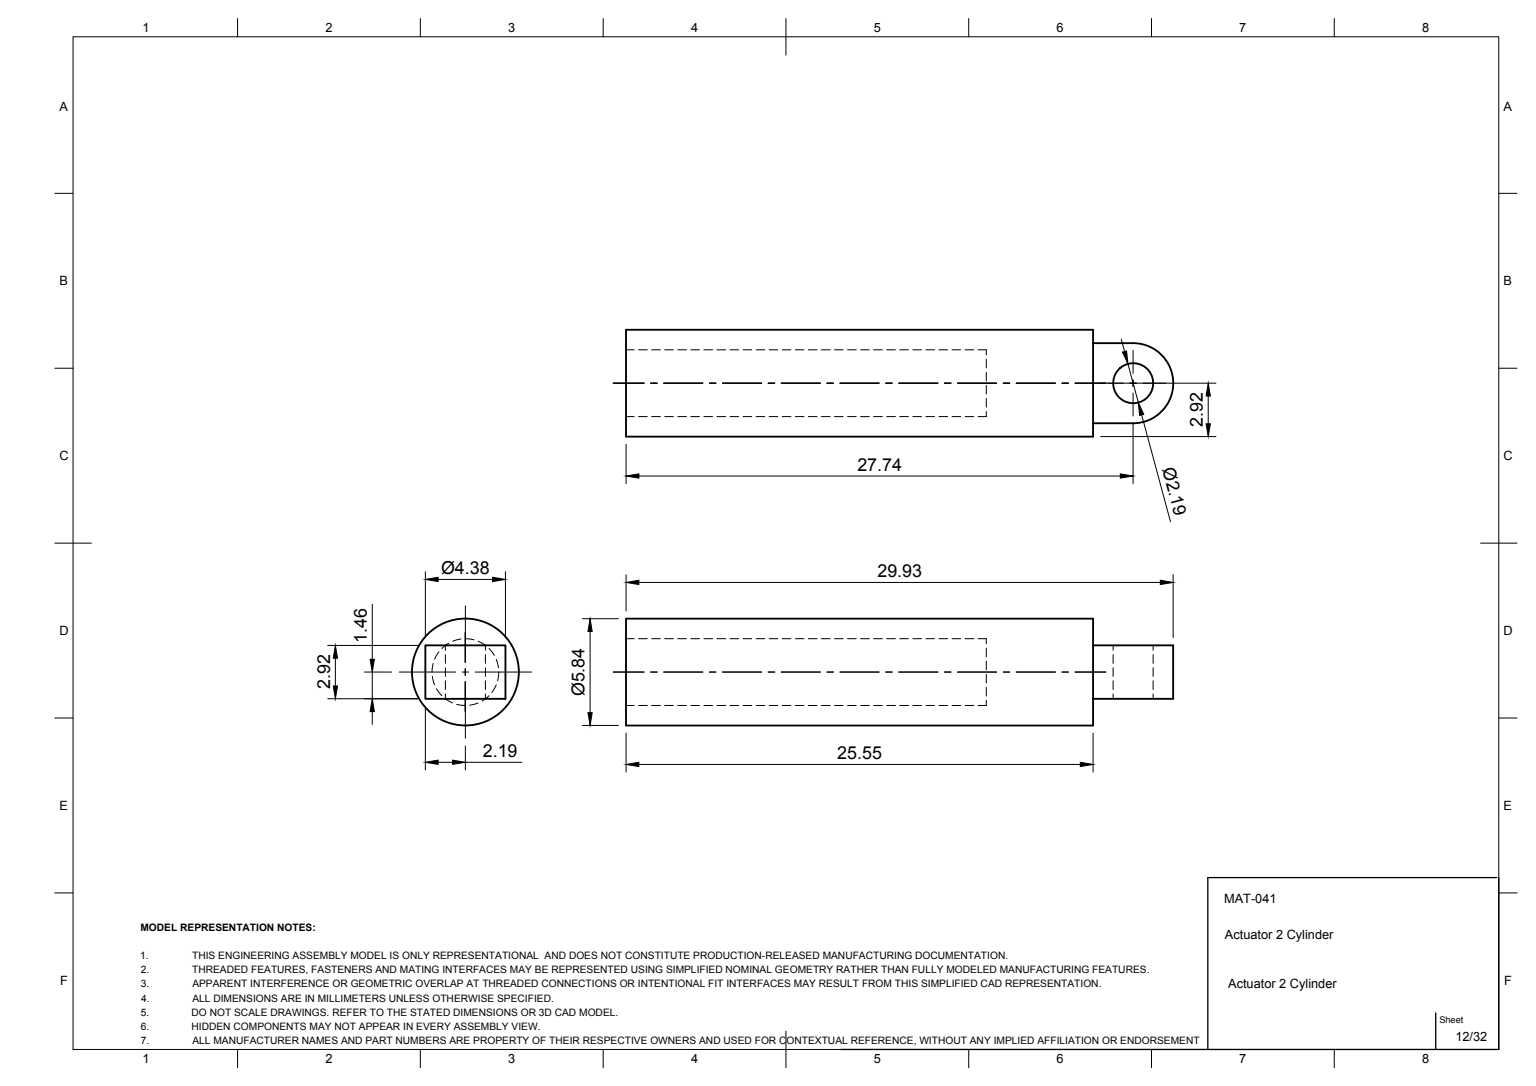
ISO-10303-21;
HEADER;
/* Generated by software containing ST-Developer
 * from STEP Tools, Inc. (www.steptools.com) 
 */

FILE_DESCRIPTION(
/* description */ ('STEP AP214'),
/* implementation_level */ '2;1');

FILE_NAME(
/* name */ 'Actuator 2 Cylinder.step',
/* time_stamp */ '2026-11-14T21:57:47-08:00',
/* author */ (''),
/* organization */ (''),
/* preprocessor_version */ 'ST-DEVELOPER v20.2',
/* originating_system */ 'Autodesk Translation Framework v15.17.0.0',
/* authorisation */ '');

FILE_SCHEMA (('AUTOMOTIVE_DESIGN { 1 0 10303 214 3 1 1 }'));
ENDSEC;

DATA;
#10=MECHANICAL_DESIGN_GEOMETRIC_PRESENTATION_REPRESENTATION('',(#252),#13199);
#216=SHAPE_REPRESENTATION_RELATIONSHIP('SRR','None',#13285,#234);
#234=ADVANCED_BREP_SHAPE_REPRESENTATION('',(#270),#13181);
#252=STYLED_ITEM('',(#13409),#270);
#270=MANIFOLD_SOLID_BREP('Body1',#6847);
#324=FACE_BOUND('',#2433,.T.);
#325=FACE_BOUND('',#2435,.T.);
#326=FACE_BOUND('',#2437,.T.);
#327=FACE_BOUND('',#2440,.T.);
#485=PLANE('',#7464);
#486=PLANE('',#7465);
#487=PLANE('',#7466);
#488=PLANE('',#7468);
#489=PLANE('',#7469);
#490=PLANE('',#7471);
#491=PLANE('',#7473);
#860=LINE('',#11592,#1378);
#861=LINE('',#11598,#1379);
#862=LINE('',#11604,#1380);
#863=LINE('',#11609,#1381);
#864=LINE('',#11611,#1382);
#865=LINE('',#11613,#1383);
#866=LINE('',#11614,#1384);
#867=LINE('',#11620,#1385);
#868=LINE('',#11621,#1386);
#869=LINE('',#11624,#1387);
#870=LINE('',#11625,#1388);
#871=LINE('',#11628,#1389);
#872=LINE('',#11631,#1390);
#1378=VECTOR('',#8873,1.825);
#1379=VECTOR('',#8880,1.095);
#1380=VECTOR('',#8887,2.92);
#1381=VECTOR('',#8892,1000.);
#1382=VECTOR('',#8893,1000.);
#1383=VECTOR('',#8894,1000.);
#1384=VECTOR('',#8895,1000.);
#1385=VECTOR('',#8902,1000.);
#1386=VECTOR('',#8903,1000.);
#1387=VECTOR('',#8906,1000.);
#1388=VECTOR('',#8907,1000.);
#1389=VECTOR('',#8910,1000.);
#1390=VECTOR('',#8915,1000.);
#1730=CYLINDRICAL_SURFACE('',#7455,1.825);
#1731=CYLINDRICAL_SURFACE('',#7458,1.095);
#1732=CYLINDRICAL_SURFACE('',#7461,2.92);
#1733=CYLINDRICAL_SURFACE('',#7472,2.19);
#1998=FACE_OUTER_BOUND('',#2429,.T.);
#1999=FACE_OUTER_BOUND('',#2430,.T.);
#2000=FACE_OUTER_BOUND('',#2431,.T.);
#2001=FACE_OUTER_BOUND('',#2432,.T.);
#2002=FACE_OUTER_BOUND('',#2434,.T.);
#2003=FACE_OUTER_BOUND('',#2436,.T.);
#2004=FACE_OUTER_BOUND('',#2438,.T.);
#2005=FACE_OUTER_BOUND('',#2439,.T.);
#2006=FACE_OUTER_BOUND('',#2441,.T.);
#2007=FACE_OUTER_BOUND('',#2442,.T.);
#2008=FACE_OUTER_BOUND('',#2443,.T.);
#2429=EDGE_LOOP('',(#5550,#5551,#5552,#5553));
#2430=EDGE_LOOP('',(#5554,#5555,#5556,#5557));
#2431=EDGE_LOOP('',(#5558,#5559,#5560,#5561));
#2432=EDGE_LOOP('',(#5562));
#2433=EDGE_LOOP('',(#5563,#5564,#5565,#5566));
#2434=EDGE_LOOP('',(#5567));
#2435=EDGE_LOOP('',(#5568));
#2436=EDGE_LOOP('',(#5569,#5570,#5571,#5572));
#2437=EDGE_LOOP('',(#5573));
#2438=EDGE_LOOP('',(#5574,#5575,#5576,#5577));
#2439=EDGE_LOOP('',(#5578,#5579,#5580,#5581));
#2440=EDGE_LOOP('',(#5582));
#2441=EDGE_LOOP('',(#5583,#5584,#5585,#5586));
#2442=EDGE_LOOP('',(#5587,#5588,#5589,#5590));
#2443=EDGE_LOOP('',(#5591));
#2861=CIRCLE('',#7456,1.825);
#2862=CIRCLE('',#7457,1.825);
#2863=CIRCLE('',#7459,1.095);
#2864=CIRCLE('',#7460,1.095);
#2865=CIRCLE('',#7462,2.92);
#2866=CIRCLE('',#7463,2.92);
#2867=CIRCLE('',#7467,2.19);
#2868=CIRCLE('',#7470,2.19);
#3318=VERTEX_POINT('',#11589);
#3319=VERTEX_POINT('',#11591);
#3320=VERTEX_POINT('',#11595);
#3321=VERTEX_POINT('',#11597);
#3322=VERTEX_POINT('',#11601);
#3323=VERTEX_POINT('',#11603);
#3324=VERTEX_POINT('',#11607);
#3325=VERTEX_POINT('',#11608);
#3326=VERTEX_POINT('',#11610);
#3327=VERTEX_POINT('',#11612);
#3328=VERTEX_POINT('',#11617);
#3329=VERTEX_POINT('',#11618);
#3330=VERTEX_POINT('',#11623);
#3331=VERTEX_POINT('',#11627);
#4112=EDGE_CURVE('',#3318,#3318,#2861,.T.);
#4113=EDGE_CURVE('',#3318,#3319,#860,.T.);
#4114=EDGE_CURVE('',#3319,#3319,#2862,.T.);
#4115=EDGE_CURVE('',#3320,#3320,#2863,.T.);
#4116=EDGE_CURVE('',#3320,#3321,#861,.T.);
#4117=EDGE_CURVE('',#3321,#3321,#2864,.T.);
#4118=EDGE_CURVE('',#3322,#3322,#2865,.T.);
#4119=EDGE_CURVE('',#3322,#3323,#862,.T.);
#4120=EDGE_CURVE('',#3323,#3323,#2866,.T.);
#4121=EDGE_CURVE('',#3324,#3325,#863,.T.);
#4122=EDGE_CURVE('',#3326,#3324,#864,.T.);
#4123=EDGE_CURVE('',#3327,#3326,#865,.T.);
#4124=EDGE_CURVE('',#3325,#3327,#866,.T.);
#4125=EDGE_CURVE('',#3328,#3329,#2867,.T.);
#4126=EDGE_CURVE('',#3329,#3324,#867,.T.);
#4127=EDGE_CURVE('',#3328,#3325,#868,.T.);
#4128=EDGE_CURVE('',#3330,#3327,#869,.T.);
#4129=EDGE_CURVE('',#3330,#3328,#870,.T.);
#4130=EDGE_CURVE('',#3331,#3326,#871,.T.);
#4131=EDGE_CURVE('',#3331,#3330,#2868,.T.);
#4132=EDGE_CURVE('',#3329,#3331,#872,.T.);
#5550=ORIENTED_EDGE('',*,*,#4112,.F.);
#5551=ORIENTED_EDGE('',*,*,#4113,.T.);
#5552=ORIENTED_EDGE('',*,*,#4114,.T.);
#5553=ORIENTED_EDGE('',*,*,#4113,.F.);
#5554=ORIENTED_EDGE('',*,*,#4115,.F.);
#5555=ORIENTED_EDGE('',*,*,#4116,.T.);
#5556=ORIENTED_EDGE('',*,*,#4117,.T.);
#5557=ORIENTED_EDGE('',*,*,#4116,.F.);
#5558=ORIENTED_EDGE('',*,*,#4118,.T.);
#5559=ORIENTED_EDGE('',*,*,#4119,.T.);
#5560=ORIENTED_EDGE('',*,*,#4120,.F.);
#5561=ORIENTED_EDGE('',*,*,#4119,.F.);
#5562=ORIENTED_EDGE('',*,*,#4118,.F.);
#5563=ORIENTED_EDGE('',*,*,#4121,.F.);
#5564=ORIENTED_EDGE('',*,*,#4122,.F.);
#5565=ORIENTED_EDGE('',*,*,#4123,.F.);
#5566=ORIENTED_EDGE('',*,*,#4124,.F.);
#5567=ORIENTED_EDGE('',*,*,#4120,.T.);
#5568=ORIENTED_EDGE('',*,*,#4114,.F.);
#5569=ORIENTED_EDGE('',*,*,#4125,.T.);
#5570=ORIENTED_EDGE('',*,*,#4126,.T.);
#5571=ORIENTED_EDGE('',*,*,#4121,.T.);
#5572=ORIENTED_EDGE('',*,*,#4127,.F.);
#5573=ORIENTED_EDGE('',*,*,#4115,.T.);
#5574=ORIENTED_EDGE('',*,*,#4128,.F.);
#5575=ORIENTED_EDGE('',*,*,#4129,.T.);
#5576=ORIENTED_EDGE('',*,*,#4127,.T.);
#5577=ORIENTED_EDGE('',*,*,#4124,.T.);
#5578=ORIENTED_EDGE('',*,*,#4130,.F.);
#5579=ORIENTED_EDGE('',*,*,#4131,.T.);
#5580=ORIENTED_EDGE('',*,*,#4128,.T.);
#5581=ORIENTED_EDGE('',*,*,#4123,.T.);
#5582=ORIENTED_EDGE('',*,*,#4117,.F.);
#5583=ORIENTED_EDGE('',*,*,#4126,.F.);
#5584=ORIENTED_EDGE('',*,*,#4132,.T.);
#5585=ORIENTED_EDGE('',*,*,#4130,.T.);
#5586=ORIENTED_EDGE('',*,*,#4122,.T.);
#5587=ORIENTED_EDGE('',*,*,#4129,.F.);
#5588=ORIENTED_EDGE('',*,*,#4131,.F.);
#5589=ORIENTED_EDGE('',*,*,#4132,.F.);
#5590=ORIENTED_EDGE('',*,*,#4125,.F.);
#5591=ORIENTED_EDGE('',*,*,#4112,.T.);
#6650=ADVANCED_FACE('',(#1998),#1730,.F.);
#6651=ADVANCED_FACE('',(#1999),#1731,.F.);
#6652=ADVANCED_FACE('',(#2000),#1732,.T.);
#6653=ADVANCED_FACE('',(#2001,#324),#485,.F.);
#6654=ADVANCED_FACE('',(#2002,#325),#486,.T.);
#6655=ADVANCED_FACE('',(#2003,#326),#487,.F.);
#6656=ADVANCED_FACE('',(#2004),#488,.F.);
#6657=ADVANCED_FACE('',(#2005,#327),#489,.F.);
#6658=ADVANCED_FACE('',(#2006),#490,.F.);
#6659=ADVANCED_FACE('',(#2007),#1733,.T.);
#6660=ADVANCED_FACE('',(#2008),#491,.T.);
#6847=CLOSED_SHELL('',(#6650,#6651,#6652,#6653,#6654,#6655,#6656,#6657,
#6658,#6659,#6660));
#7454=AXIS2_PLACEMENT_3D('',#11587,#8867,#8868);
#7455=AXIS2_PLACEMENT_3D('',#11588,#8869,#8870);
#7456=AXIS2_PLACEMENT_3D('',#11590,#8871,#8872);
#7457=AXIS2_PLACEMENT_3D('',#11593,#8874,#8875);
#7458=AXIS2_PLACEMENT_3D('',#11594,#8876,#8877);
#7459=AXIS2_PLACEMENT_3D('',#11596,#8878,#8879);
#7460=AXIS2_PLACEMENT_3D('',#11599,#8881,#8882);
#7461=AXIS2_PLACEMENT_3D('',#11600,#8883,#8884);
#7462=AXIS2_PLACEMENT_3D('',#11602,#8885,#8886);
#7463=AXIS2_PLACEMENT_3D('',#11605,#8888,#8889);
#7464=AXIS2_PLACEMENT_3D('',#11606,#8890,#8891);
#7465=AXIS2_PLACEMENT_3D('',#11615,#8896,#8897);
#7466=AXIS2_PLACEMENT_3D('',#11616,#8898,#8899);
#7467=AXIS2_PLACEMENT_3D('',#11619,#8900,#8901);
#7468=AXIS2_PLACEMENT_3D('',#11622,#8904,#8905);
#7469=AXIS2_PLACEMENT_3D('',#11626,#8908,#8909);
#7470=AXIS2_PLACEMENT_3D('',#11629,#8911,#8912);
#7471=AXIS2_PLACEMENT_3D('',#11630,#8913,#8914);
#7472=AXIS2_PLACEMENT_3D('',#11632,#8916,#8917);
#7473=AXIS2_PLACEMENT_3D('',#11633,#8918,#8919);
#8867=DIRECTION('axis',(0.,0.,1.));
#8868=DIRECTION('refdir',(1.,0.,0.));
#8869=DIRECTION('center_axis',(0.,0.,1.));
#8870=DIRECTION('ref_axis',(1.,0.,0.));
#8871=DIRECTION('center_axis',(0.,0.,1.));
#8872=DIRECTION('ref_axis',(1.,0.,0.));
#8873=DIRECTION('',(0.,0.,1.));
#8874=DIRECTION('center_axis',(0.,0.,1.));
#8875=DIRECTION('ref_axis',(1.,0.,0.));
#8876=DIRECTION('center_axis',(1.,-1.0842021724855E-16,0.));
#8877=DIRECTION('ref_axis',(1.0842021724855E-16,1.,0.));
#8878=DIRECTION('center_axis',(1.,-7.2280144832367E-17,0.));
#8879=DIRECTION('ref_axis',(7.2280144832367E-17,1.,0.));
#8880=DIRECTION('',(1.,-1.0842021724855E-16,0.));
#8881=DIRECTION('center_axis',(1.,-1.0842021724855E-16,0.));
#8882=DIRECTION('ref_axis',(1.0842021724855E-16,1.,0.));
#8883=DIRECTION('center_axis',(0.,0.,-1.));
#8884=DIRECTION('ref_axis',(-1.,0.,0.));
#8885=DIRECTION('center_axis',(0.,0.,1.));
#8886=DIRECTION('ref_axis',(1.,0.,0.));
#8887=DIRECTION('',(0.,0.,1.));
#8888=DIRECTION('center_axis',(0.,0.,1.));
#8889=DIRECTION('ref_axis',(1.,0.,0.));
#8890=DIRECTION('center_axis',(0.,0.,1.));
#8891=DIRECTION('ref_axis',(1.,0.,0.));
#8892=DIRECTION('',(7.2280144832367E-17,1.,0.));
#8893=DIRECTION('',(-1.,0.,0.));
#8894=DIRECTION('',(-1.44560289664734E-16,-1.,0.));
#8895=DIRECTION('',(1.,0.,0.));
#8896=DIRECTION('center_axis',(0.,0.,1.));
#8897=DIRECTION('ref_axis',(1.,0.,0.));
#8898=DIRECTION('center_axis',(1.,-7.2280144832367E-17,0.));
#8899=DIRECTION('ref_axis',(7.2280144832367E-17,1.,0.));
#8900=DIRECTION('center_axis',(-1.,7.2280144832367E-17,0.));
#8901=DIRECTION('ref_axis',(7.2280144832367E-17,1.,0.));
#8902=DIRECTION('',(0.,0.,1.));
#8903=DIRECTION('',(0.,0.,1.));
#8904=DIRECTION('center_axis',(0.,-1.,0.));
#8905=DIRECTION('ref_axis',(0.,0.,-1.));
#8906=DIRECTION('',(0.,0.,1.));
#8907=DIRECTION('',(-1.,0.,0.));
#8908=DIRECTION('center_axis',(-1.,1.44560289664734E-16,0.));
#8909=DIRECTION('ref_axis',(-1.44560289664734E-16,-1.,0.));
#8910=DIRECTION('',(0.,0.,1.));
#8911=DIRECTION('center_axis',(1.,-1.44560289664734E-16,0.));
#8912=DIRECTION('ref_axis',(-1.44560289664734E-16,-1.,0.));
#8913=DIRECTION('center_axis',(0.,1.,0.));
#8914=DIRECTION('ref_axis',(0.,0.,1.));
#8915=DIRECTION('',(1.,0.,0.));
#8916=DIRECTION('center_axis',(-1.,0.,0.));
#8917=DIRECTION('ref_axis',(0.,1.22464679914735E-16,-1.));
#8918=DIRECTION('center_axis',(0.,0.,1.));
#8919=DIRECTION('ref_axis',(1.,0.,0.));
#11587=CARTESIAN_POINT('',(0.,0.,0.));
#11588=CARTESIAN_POINT('Origin',(0.,0.,9.72414336253035));
#11589=CARTESIAN_POINT('',(-1.825,-2.23498040844392E-16,9.72414336253035));
#11590=CARTESIAN_POINT('Origin',(0.,0.,9.72414336253035));
#11591=CARTESIAN_POINT('',(-1.825,-2.23498040844392E-16,29.4341433625304));
#11592=CARTESIAN_POINT('',(-1.825,-2.23498040844392E-16,9.72414336253035));
#11593=CARTESIAN_POINT('Origin',(0.,0.,29.4341433625304));
#11594=CARTESIAN_POINT('Origin',(-2.92,4.33680868994202E-16,1.69414336253035));
#11595=CARTESIAN_POINT('',(-1.46,-1.095,1.69414336253035));
#11596=CARTESIAN_POINT('Origin',(-1.46,4.33680868994202E-16,1.69414336253035));
#11597=CARTESIAN_POINT('',(1.46,-1.095,1.69414336253035));
#11598=CARTESIAN_POINT('',(-2.92,-1.095,1.69414336253035));
#11599=CARTESIAN_POINT('Origin',(1.46,0.,1.69414336253035));
#11600=CARTESIAN_POINT('Origin',(0.,0.,29.4341433625304));
#11601=CARTESIAN_POINT('',(2.92,-3.57596865351027E-16,3.88414336253035));
#11602=CARTESIAN_POINT('Origin',(0.,0.,3.88414336253035));
#11603=CARTESIAN_POINT('',(2.92,-3.57596865351027E-16,29.4341433625304));
#11604=CARTESIAN_POINT('',(2.92,-3.57596865351027E-16,29.4341433625304));
#11605=CARTESIAN_POINT('Origin',(0.,0.,29.4341433625304));
#11606=CARTESIAN_POINT('Origin',(0.,0.,3.88414336253035));
#11607=CARTESIAN_POINT('',(-1.46,-2.19,3.88414336253035));
#11608=CARTESIAN_POINT('',(-1.46,2.19,3.88414336253035));
#11609=CARTESIAN_POINT('',(-1.46,2.19,3.88414336253035));
#11610=CARTESIAN_POINT('',(1.46,-2.19,3.88414336253035));
#11611=CARTESIAN_POINT('',(1.46,-2.19,3.88414336253035));
#11612=CARTESIAN_POINT('',(1.46,2.19,3.88414336253035));
#11613=CARTESIAN_POINT('',(1.46,2.19,3.88414336253035));
#11614=CARTESIAN_POINT('',(1.46,2.19,3.88414336253035));
#11615=CARTESIAN_POINT('Origin',(0.,0.,29.4341433625304));
#11616=CARTESIAN_POINT('Origin',(-1.46,2.19,-0.495856637469653));
#11617=CARTESIAN_POINT('',(-1.46,2.19,1.69414336253035));
#11618=CARTESIAN_POINT('',(-1.46,-2.19,1.69414336253035));
#11619=CARTESIAN_POINT('Origin',(-1.46,0.,1.69414336253035));
#11620=CARTESIAN_POINT('',(-1.46,-2.19,-0.495856637469653));
#11621=CARTESIAN_POINT('',(-1.46,2.19,-0.495856637469653));
#11622=CARTESIAN_POINT('Origin',(1.46,2.19,-0.495856637469653));
#11623=CARTESIAN_POINT('',(1.46,2.19,1.69414336253035));
#11624=CARTESIAN_POINT('',(1.46,2.19,-0.495856637469653));
#11625=CARTESIAN_POINT('',(-1.46,2.19,1.69414336253035));
#11626=CARTESIAN_POINT('Origin',(1.46,2.19,-0.495856637469653));
#11627=CARTESIAN_POINT('',(1.46,-2.19,1.69414336253035));
#11628=CARTESIAN_POINT('',(1.46,-2.19,-0.495856637469653));
#11629=CARTESIAN_POINT('Origin',(1.46,0.,1.69414336253035));
#11630=CARTESIAN_POINT('Origin',(1.46,-2.19,-0.495856637469653));
#11631=CARTESIAN_POINT('',(1.46,-2.19,1.69414336253035));
#11632=CARTESIAN_POINT('Origin',(0.,0.,1.69414336253035));
#11633=CARTESIAN_POINT('Origin',(0.,0.,9.72414336253035));
#13155=UNCERTAINTY_MEASURE_WITH_UNIT(LENGTH_MEASURE(0.01),#13200,
'DISTANCE_ACCURACY_VALUE',
'Maximum model space distance between geometric entities at asserted c
onnectivities');
#13173=UNCERTAINTY_MEASURE_WITH_UNIT(LENGTH_MEASURE(0.01),#13200,
'DISTANCE_ACCURACY_VALUE',
'Maximum model space distance between geometric entities at asserted c
onnectivities');
#13181=(
GEOMETRIC_REPRESENTATION_CONTEXT(3)
GLOBAL_UNCERTAINTY_ASSIGNED_CONTEXT((#13155))
GLOBAL_UNIT_ASSIGNED_CONTEXT((#13200,#13202,#13203))
REPRESENTATION_CONTEXT('','3D')
);
#13199=(
GEOMETRIC_REPRESENTATION_CONTEXT(3)
GLOBAL_UNCERTAINTY_ASSIGNED_CONTEXT((#13173))
GLOBAL_UNIT_ASSIGNED_CONTEXT((#13200,#13202,#13203))
REPRESENTATION_CONTEXT('','3D')
);
#13200=(
LENGTH_UNIT()
NAMED_UNIT(*)
SI_UNIT(.MILLI.,.METRE.)
);
#13202=(
NAMED_UNIT(*)
PLANE_ANGLE_UNIT()
SI_UNIT($,.RADIAN.)
);
#13203=(
NAMED_UNIT(*)
SI_UNIT($,.STERADIAN.)
SOLID_ANGLE_UNIT()
);
#13211=SHAPE_DEFINITION_REPRESENTATION(#13236,#13285);
#13236=PRODUCT_DEFINITION_SHAPE('',$,#13311);
#13285=SHAPE_REPRESENTATION('',(#7454),#13181);
#13303=PRODUCT_DEFINITION_CONTEXT('part definition',#13380,'design');
#13311=PRODUCT_DEFINITION('Actuator 2 Cylinder','Actuator 2 Cylinder',#13336,
#13303);
#13336=PRODUCT_DEFINITION_FORMATION('',$,#13389);
#13380=APPLICATION_CONTEXT(
'Core Data for Automotive Mechanical Design Process');
#13381=PRODUCT_CONTEXT('part definition',#13380,'mechanical');
#13389=PRODUCT('Actuator 2 Cylinder','Actuator 2 Cylinder',$,(#13381));
#13409=PRESENTATION_STYLE_ASSIGNMENT((#13414));
#13414=SURFACE_STYLE_USAGE(.BOTH.,#13419);
#13419=SURFACE_SIDE_STYLE('',(#13424));
#13424=SURFACE_STYLE_FILL_AREA(#13429);
#13429=FILL_AREA_STYLE('Opaque(61,176,222)',(#13434));
#13434=FILL_AREA_STYLE_COLOUR('Opaque(61,176,222)',#13439);
#13439=COLOUR_RGB('Opaque(61,176,222)',0.23921568627451,0.690196078431373,
0.870588235294118);
ENDSEC;
END-ISO-10303-21;
